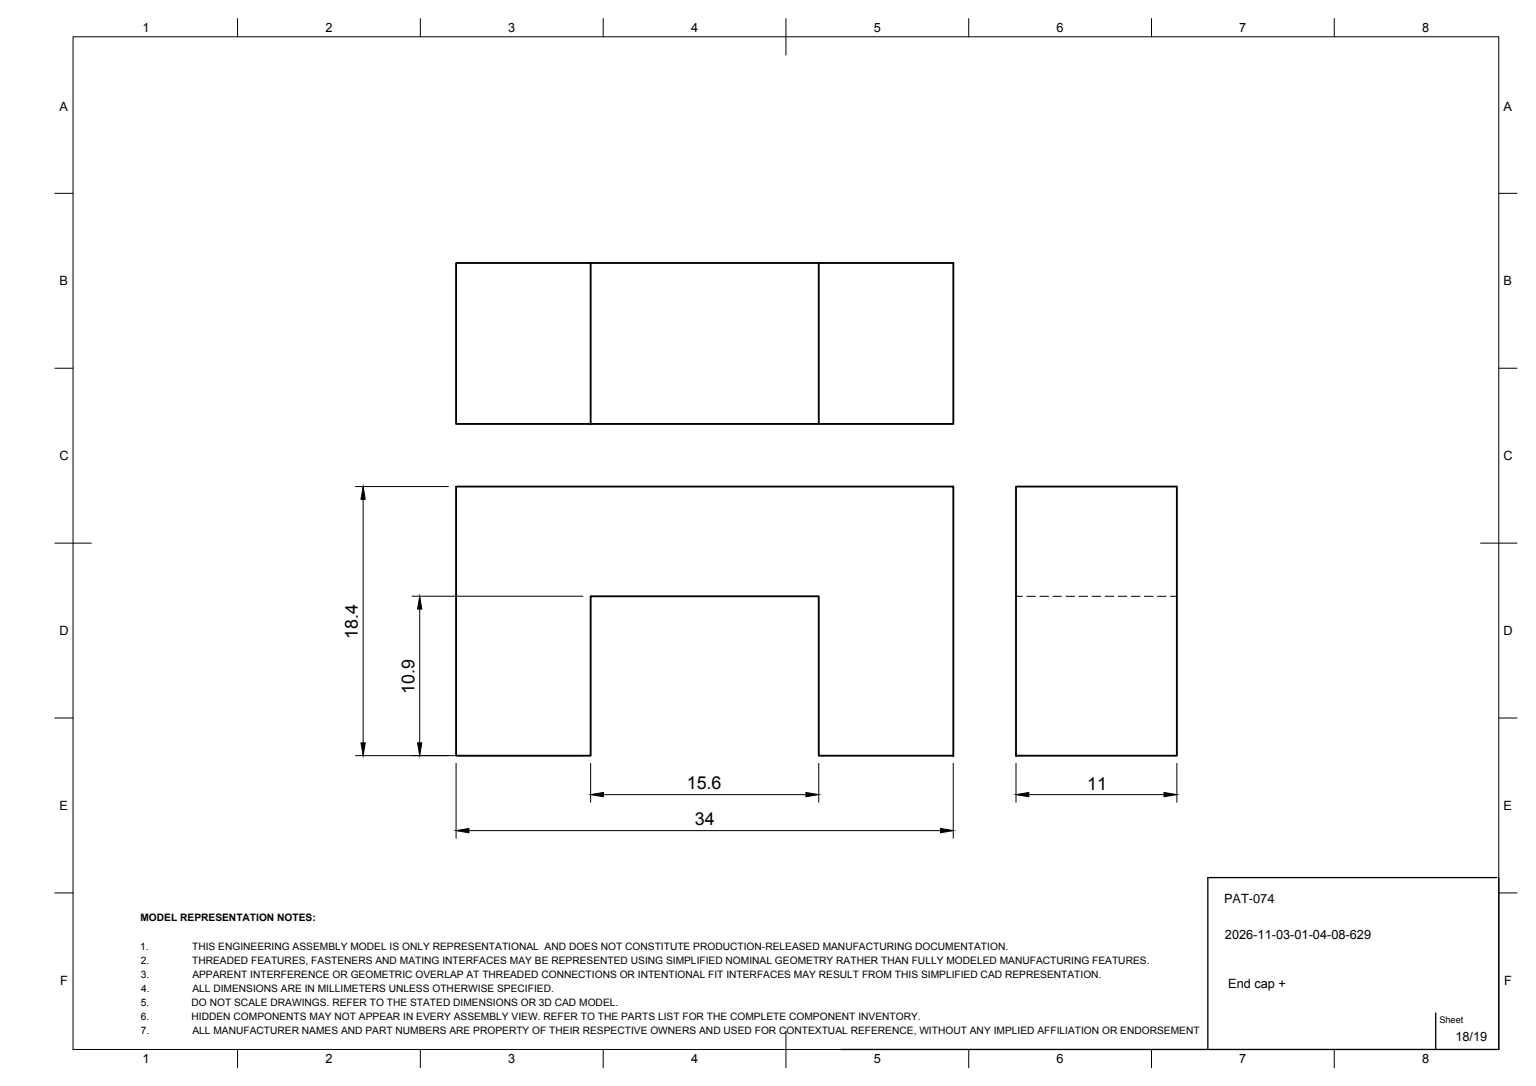
ISO-10303-21;
HEADER;
/* Generated by software containing ST-Developer
 * from STEP Tools, Inc. (www.steptools.com) 
 */

FILE_DESCRIPTION(
/* description */ ('Manual rail carriage with stops'),
/* implementation_level */ '2;1');

FILE_NAME(
/* name */ 'End cap +.step',
/* time_stamp */ '2026-10-27T18:54:27-07:00',
/* author */ (''),
/* organization */ (''),
/* preprocessor_version */ 'ST-DEVELOPER v20.2',
/* originating_system */ 'Autodesk Translation Framework v15.17.0.0',
/* authorisation */ '');

FILE_SCHEMA (('AUTOMOTIVE_DESIGN { 1 0 10303 214 3 1 1 }'));
ENDSEC;

DATA;
#10=MECHANICAL_DESIGN_GEOMETRIC_PRESENTATION_REPRESENTATION('',(#283),#8499);
#247=SHAPE_REPRESENTATION_RELATIONSHIP('SRR','None',#8612,#265);
#265=ADVANCED_BREP_SHAPE_REPRESENTATION('',(#299),#8491);
#283=STYLED_ITEM('',(#8781),#299);
#299=MANIFOLD_SOLID_BREP('Body1',#4953);
#523=PLANE('',#5454);
#524=PLANE('',#5455);
#525=PLANE('',#5456);
#526=PLANE('',#5457);
#527=PLANE('',#5458);
#528=PLANE('',#5459);
#529=PLANE('',#5460);
#530=PLANE('',#5461);
#531=PLANE('',#5462);
#532=PLANE('',#5463);
#763=FACE_OUTER_BOUND('',#1083,.T.);
#764=FACE_OUTER_BOUND('',#1084,.T.);
#765=FACE_OUTER_BOUND('',#1085,.T.);
#766=FACE_OUTER_BOUND('',#1086,.T.);
#767=FACE_OUTER_BOUND('',#1087,.T.);
#768=FACE_OUTER_BOUND('',#1088,.T.);
#769=FACE_OUTER_BOUND('',#1089,.T.);
#770=FACE_OUTER_BOUND('',#1090,.T.);
#771=FACE_OUTER_BOUND('',#1091,.T.);
#772=FACE_OUTER_BOUND('',#1092,.T.);
#1083=EDGE_LOOP('',(#4300,#4301,#4302,#4303));
#1084=EDGE_LOOP('',(#4304,#4305,#4306,#4307));
#1085=EDGE_LOOP('',(#4308,#4309,#4310,#4311));
#1086=EDGE_LOOP('',(#4312,#4313,#4314,#4315));
#1087=EDGE_LOOP('',(#4316,#4317,#4318,#4319));
#1088=EDGE_LOOP('',(#4320,#4321,#4322,#4323));
#1089=EDGE_LOOP('',(#4324,#4325,#4326,#4327));
#1090=EDGE_LOOP('',(#4328,#4329,#4330,#4331));
#1091=EDGE_LOOP('',(#4332,#4333,#4334,#4335,#4336,#4337,#4338,#4339));
#1092=EDGE_LOOP('',(#4340,#4341,#4342,#4343,#4344,#4345,#4346,#4347));
#1561=LINE('',#8054,#2061);
#1562=LINE('',#8056,#2062);
#1563=LINE('',#8058,#2063);
#1564=LINE('',#8059,#2064);
#1565=LINE('',#8062,#2065);
#1566=LINE('',#8064,#2066);
#1567=LINE('',#8065,#2067);
#1568=LINE('',#8068,#2068);
#1569=LINE('',#8070,#2069);
#1570=LINE('',#8071,#2070);
#1571=LINE('',#8074,#2071);
#1572=LINE('',#8076,#2072);
#1573=LINE('',#8077,#2073);
#1574=LINE('',#8080,#2074);
#1575=LINE('',#8082,#2075);
#1576=LINE('',#8083,#2076);
#1577=LINE('',#8086,#2077);
#1578=LINE('',#8088,#2078);
#1579=LINE('',#8089,#2079);
#1580=LINE('',#8092,#2080);
#1581=LINE('',#8094,#2081);
#1582=LINE('',#8095,#2082);
#1583=LINE('',#8097,#2083);
#1584=LINE('',#8098,#2084);
#2061=VECTOR('',#6596,1.);
#2062=VECTOR('',#6597,1.);
#2063=VECTOR('',#6598,1.);
#2064=VECTOR('',#6599,1.);
#2065=VECTOR('',#6602,1.);
#2066=VECTOR('',#6603,1.);
#2067=VECTOR('',#6604,1.);
#2068=VECTOR('',#6607,1.);
#2069=VECTOR('',#6608,1.);
#2070=VECTOR('',#6609,1.);
#2071=VECTOR('',#6612,1.);
#2072=VECTOR('',#6613,1.);
#2073=VECTOR('',#6614,1.);
#2074=VECTOR('',#6617,1.);
#2075=VECTOR('',#6618,1.);
#2076=VECTOR('',#6619,1.);
#2077=VECTOR('',#6622,1.);
#2078=VECTOR('',#6623,1.);
#2079=VECTOR('',#6624,1.);
#2080=VECTOR('',#6627,1.);
#2081=VECTOR('',#6628,1.);
#2082=VECTOR('',#6629,1.);
#2083=VECTOR('',#6632,1.);
#2084=VECTOR('',#6633,1.);
#2623=VERTEX_POINT('',#8052);
#2624=VERTEX_POINT('',#8053);
#2625=VERTEX_POINT('',#8055);
#2626=VERTEX_POINT('',#8057);
#2627=VERTEX_POINT('',#8061);
#2628=VERTEX_POINT('',#8063);
#2629=VERTEX_POINT('',#8067);
#2630=VERTEX_POINT('',#8069);
#2631=VERTEX_POINT('',#8073);
#2632=VERTEX_POINT('',#8075);
#2633=VERTEX_POINT('',#8079);
#2634=VERTEX_POINT('',#8081);
#2635=VERTEX_POINT('',#8085);
#2636=VERTEX_POINT('',#8087);
#2637=VERTEX_POINT('',#8091);
#2638=VERTEX_POINT('',#8093);
#3198=EDGE_CURVE('',#2623,#2624,#1561,.T.);
#3199=EDGE_CURVE('',#2624,#2625,#1562,.T.);
#3200=EDGE_CURVE('',#2626,#2625,#1563,.T.);
#3201=EDGE_CURVE('',#2623,#2626,#1564,.T.);
#3202=EDGE_CURVE('',#2627,#2623,#1565,.T.);
#3203=EDGE_CURVE('',#2628,#2626,#1566,.T.);
#3204=EDGE_CURVE('',#2627,#2628,#1567,.T.);
#3205=EDGE_CURVE('',#2629,#2627,#1568,.T.);
#3206=EDGE_CURVE('',#2630,#2628,#1569,.T.);
#3207=EDGE_CURVE('',#2629,#2630,#1570,.T.);
#3208=EDGE_CURVE('',#2631,#2629,#1571,.T.);
#3209=EDGE_CURVE('',#2632,#2630,#1572,.T.);
#3210=EDGE_CURVE('',#2631,#2632,#1573,.T.);
#3211=EDGE_CURVE('',#2633,#2631,#1574,.T.);
#3212=EDGE_CURVE('',#2634,#2632,#1575,.T.);
#3213=EDGE_CURVE('',#2633,#2634,#1576,.T.);
#3214=EDGE_CURVE('',#2635,#2633,#1577,.T.);
#3215=EDGE_CURVE('',#2636,#2634,#1578,.T.);
#3216=EDGE_CURVE('',#2635,#2636,#1579,.T.);
#3217=EDGE_CURVE('',#2637,#2635,#1580,.T.);
#3218=EDGE_CURVE('',#2638,#2636,#1581,.T.);
#3219=EDGE_CURVE('',#2637,#2638,#1582,.T.);
#3220=EDGE_CURVE('',#2624,#2637,#1583,.T.);
#3221=EDGE_CURVE('',#2625,#2638,#1584,.T.);
#4300=ORIENTED_EDGE('',*,*,#3198,.T.);
#4301=ORIENTED_EDGE('',*,*,#3199,.T.);
#4302=ORIENTED_EDGE('',*,*,#3200,.F.);
#4303=ORIENTED_EDGE('',*,*,#3201,.F.);
#4304=ORIENTED_EDGE('',*,*,#3202,.T.);
#4305=ORIENTED_EDGE('',*,*,#3201,.T.);
#4306=ORIENTED_EDGE('',*,*,#3203,.F.);
#4307=ORIENTED_EDGE('',*,*,#3204,.F.);
#4308=ORIENTED_EDGE('',*,*,#3205,.T.);
#4309=ORIENTED_EDGE('',*,*,#3204,.T.);
#4310=ORIENTED_EDGE('',*,*,#3206,.F.);
#4311=ORIENTED_EDGE('',*,*,#3207,.F.);
#4312=ORIENTED_EDGE('',*,*,#3208,.T.);
#4313=ORIENTED_EDGE('',*,*,#3207,.T.);
#4314=ORIENTED_EDGE('',*,*,#3209,.F.);
#4315=ORIENTED_EDGE('',*,*,#3210,.F.);
#4316=ORIENTED_EDGE('',*,*,#3211,.T.);
#4317=ORIENTED_EDGE('',*,*,#3210,.T.);
#4318=ORIENTED_EDGE('',*,*,#3212,.F.);
#4319=ORIENTED_EDGE('',*,*,#3213,.F.);
#4320=ORIENTED_EDGE('',*,*,#3214,.T.);
#4321=ORIENTED_EDGE('',*,*,#3213,.T.);
#4322=ORIENTED_EDGE('',*,*,#3215,.F.);
#4323=ORIENTED_EDGE('',*,*,#3216,.F.);
#4324=ORIENTED_EDGE('',*,*,#3217,.T.);
#4325=ORIENTED_EDGE('',*,*,#3216,.T.);
#4326=ORIENTED_EDGE('',*,*,#3218,.F.);
#4327=ORIENTED_EDGE('',*,*,#3219,.F.);
#4328=ORIENTED_EDGE('',*,*,#3220,.T.);
#4329=ORIENTED_EDGE('',*,*,#3219,.T.);
#4330=ORIENTED_EDGE('',*,*,#3221,.F.);
#4331=ORIENTED_EDGE('',*,*,#3199,.F.);
#4332=ORIENTED_EDGE('',*,*,#3221,.T.);
#4333=ORIENTED_EDGE('',*,*,#3218,.T.);
#4334=ORIENTED_EDGE('',*,*,#3215,.T.);
#4335=ORIENTED_EDGE('',*,*,#3212,.T.);
#4336=ORIENTED_EDGE('',*,*,#3209,.T.);
#4337=ORIENTED_EDGE('',*,*,#3206,.T.);
#4338=ORIENTED_EDGE('',*,*,#3203,.T.);
#4339=ORIENTED_EDGE('',*,*,#3200,.T.);
#4340=ORIENTED_EDGE('',*,*,#3220,.F.);
#4341=ORIENTED_EDGE('',*,*,#3198,.F.);
#4342=ORIENTED_EDGE('',*,*,#3202,.F.);
#4343=ORIENTED_EDGE('',*,*,#3205,.F.);
#4344=ORIENTED_EDGE('',*,*,#3208,.F.);
#4345=ORIENTED_EDGE('',*,*,#3211,.F.);
#4346=ORIENTED_EDGE('',*,*,#3214,.F.);
#4347=ORIENTED_EDGE('',*,*,#3217,.F.);
#4862=ADVANCED_FACE('',(#763),#523,.T.);
#4863=ADVANCED_FACE('',(#764),#524,.T.);
#4864=ADVANCED_FACE('',(#765),#525,.T.);
#4865=ADVANCED_FACE('',(#766),#526,.T.);
#4866=ADVANCED_FACE('',(#767),#527,.T.);
#4867=ADVANCED_FACE('',(#768),#528,.T.);
#4868=ADVANCED_FACE('',(#769),#529,.T.);
#4869=ADVANCED_FACE('',(#770),#530,.T.);
#4870=ADVANCED_FACE('',(#771),#531,.T.);
#4871=ADVANCED_FACE('',(#772),#532,.F.);
#4953=CLOSED_SHELL('',(#4862,#4863,#4864,#4865,#4866,#4867,#4868,#4869,
#4870,#4871));
#5453=AXIS2_PLACEMENT_3D('',#8050,#6592,#6593);
#5454=AXIS2_PLACEMENT_3D('',#8051,#6594,#6595);
#5455=AXIS2_PLACEMENT_3D('',#8060,#6600,#6601);
#5456=AXIS2_PLACEMENT_3D('',#8066,#6605,#6606);
#5457=AXIS2_PLACEMENT_3D('',#8072,#6610,#6611);
#5458=AXIS2_PLACEMENT_3D('',#8078,#6615,#6616);
#5459=AXIS2_PLACEMENT_3D('',#8084,#6620,#6621);
#5460=AXIS2_PLACEMENT_3D('',#8090,#6625,#6626);
#5461=AXIS2_PLACEMENT_3D('',#8096,#6630,#6631);
#5462=AXIS2_PLACEMENT_3D('',#8099,#6634,#6635);
#5463=AXIS2_PLACEMENT_3D('',#8100,#6636,#6637);
#6592=DIRECTION('axis',(0.,0.,1.));
#6593=DIRECTION('refdir',(1.,0.,0.));
#6594=DIRECTION('center_axis',(0.,0.,1.));
#6595=DIRECTION('ref_axis',(0.,-1.,0.));
#6596=DIRECTION('',(0.,-1.,0.));
#6597=DIRECTION('',(1.,0.,0.));
#6598=DIRECTION('',(0.,-1.,0.));
#6599=DIRECTION('',(1.,0.,0.));
#6600=DIRECTION('center_axis',(0.,1.,0.));
#6601=DIRECTION('ref_axis',(0.,0.,1.));
#6602=DIRECTION('',(0.,0.,1.));
#6603=DIRECTION('',(0.,0.,1.));
#6604=DIRECTION('',(1.,0.,0.));
#6605=DIRECTION('center_axis',(0.,0.,-1.));
#6606=DIRECTION('ref_axis',(0.,1.,0.));
#6607=DIRECTION('',(0.,1.,0.));
#6608=DIRECTION('',(0.,1.,0.));
#6609=DIRECTION('',(1.,0.,0.));
#6610=DIRECTION('center_axis',(0.,-1.,0.));
#6611=DIRECTION('ref_axis',(0.,0.,-1.));
#6612=DIRECTION('',(0.,0.,-1.));
#6613=DIRECTION('',(0.,0.,-1.));
#6614=DIRECTION('',(1.,0.,0.));
#6615=DIRECTION('center_axis',(0.,0.,-1.));
#6616=DIRECTION('ref_axis',(0.,1.,0.));
#6617=DIRECTION('',(0.,1.,0.));
#6618=DIRECTION('',(0.,1.,0.));
#6619=DIRECTION('',(1.,0.,0.));
#6620=DIRECTION('center_axis',(0.,1.,0.));
#6621=DIRECTION('ref_axis',(0.,0.,1.));
#6622=DIRECTION('',(0.,0.,1.));
#6623=DIRECTION('',(0.,0.,1.));
#6624=DIRECTION('',(1.,0.,0.));
#6625=DIRECTION('center_axis',(0.,0.,-1.));
#6626=DIRECTION('ref_axis',(0.,1.,0.));
#6627=DIRECTION('',(0.,1.,0.));
#6628=DIRECTION('',(0.,1.,0.));
#6629=DIRECTION('',(1.,0.,0.));
#6630=DIRECTION('center_axis',(0.,-1.,0.));
#6631=DIRECTION('ref_axis',(0.,0.,-1.));
#6632=DIRECTION('',(0.,0.,-1.));
#6633=DIRECTION('',(0.,0.,-1.));
#6634=DIRECTION('center_axis',(1.,0.,0.));
#6635=DIRECTION('ref_axis',(0.,0.,-1.));
#6636=DIRECTION('center_axis',(1.,0.,0.));
#6637=DIRECTION('ref_axis',(0.,0.,-1.));
#8050=CARTESIAN_POINT('',(0.,0.,0.));
#8051=CARTESIAN_POINT('Origin',(1.97,1.7,2.3));
#8052=CARTESIAN_POINT('',(1.97,1.7,2.3));
#8053=CARTESIAN_POINT('',(1.97,-1.7,2.3));
#8054=CARTESIAN_POINT('',(1.97,1.7,2.3));
#8055=CARTESIAN_POINT('',(3.07,-1.7,2.3));
#8056=CARTESIAN_POINT('',(1.97,-1.7,2.3));
#8057=CARTESIAN_POINT('',(3.07,1.7,2.3));
#8058=CARTESIAN_POINT('',(3.07,1.7,2.3));
#8059=CARTESIAN_POINT('',(1.97,1.7,2.3));
#8060=CARTESIAN_POINT('Origin',(1.97,1.7,0.46));
#8061=CARTESIAN_POINT('',(1.97,1.7,0.46));
#8062=CARTESIAN_POINT('',(1.97,1.7,0.46));
#8063=CARTESIAN_POINT('',(3.07,1.7,0.46));
#8064=CARTESIAN_POINT('',(3.07,1.7,0.46));
#8065=CARTESIAN_POINT('',(1.97,1.7,0.46));
#8066=CARTESIAN_POINT('Origin',(1.97,0.78,0.46));
#8067=CARTESIAN_POINT('',(1.97,0.78,0.46));
#8068=CARTESIAN_POINT('',(1.97,0.78,0.46));
#8069=CARTESIAN_POINT('',(3.07,0.78,0.46));
#8070=CARTESIAN_POINT('',(3.07,0.78,0.46));
#8071=CARTESIAN_POINT('',(1.97,0.78,0.46));
#8072=CARTESIAN_POINT('Origin',(1.97,0.78,1.55));
#8073=CARTESIAN_POINT('',(1.97,0.78,1.55));
#8074=CARTESIAN_POINT('',(1.97,0.78,1.55));
#8075=CARTESIAN_POINT('',(3.07,0.78,1.55));
#8076=CARTESIAN_POINT('',(3.07,0.78,1.55));
#8077=CARTESIAN_POINT('',(1.97,0.78,1.55));
#8078=CARTESIAN_POINT('Origin',(1.97,-0.78,1.55));
#8079=CARTESIAN_POINT('',(1.97,-0.78,1.55));
#8080=CARTESIAN_POINT('',(1.97,-0.78,1.55));
#8081=CARTESIAN_POINT('',(3.07,-0.78,1.55));
#8082=CARTESIAN_POINT('',(3.07,-0.78,1.55));
#8083=CARTESIAN_POINT('',(1.97,-0.78,1.55));
#8084=CARTESIAN_POINT('Origin',(1.97,-0.78,0.46));
#8085=CARTESIAN_POINT('',(1.97,-0.78,0.46));
#8086=CARTESIAN_POINT('',(1.97,-0.78,0.46));
#8087=CARTESIAN_POINT('',(3.07,-0.78,0.46));
#8088=CARTESIAN_POINT('',(3.07,-0.78,0.46));
#8089=CARTESIAN_POINT('',(1.97,-0.78,0.46));
#8090=CARTESIAN_POINT('Origin',(1.97,-1.7,0.46));
#8091=CARTESIAN_POINT('',(1.97,-1.7,0.46));
#8092=CARTESIAN_POINT('',(1.97,-1.7,0.46));
#8093=CARTESIAN_POINT('',(3.07,-1.7,0.46));
#8094=CARTESIAN_POINT('',(3.07,-1.7,0.46));
#8095=CARTESIAN_POINT('',(1.97,-1.7,0.46));
#8096=CARTESIAN_POINT('Origin',(1.97,-1.7,2.3));
#8097=CARTESIAN_POINT('',(1.97,-1.7,2.3));
#8098=CARTESIAN_POINT('',(3.07,-1.7,2.3));
#8099=CARTESIAN_POINT('Origin',(3.07,0.,1.38));
#8100=CARTESIAN_POINT('Origin',(1.97,0.,1.38));
#8468=UNCERTAINTY_MEASURE_WITH_UNIT(LENGTH_MEASURE(0.001),#8500,
'DISTANCE_ACCURACY_VALUE',
'Maximum model space distance between geometric entities at asserted c
onnectivities');
#8476=UNCERTAINTY_MEASURE_WITH_UNIT(LENGTH_MEASURE(0.001),#8500,
'DISTANCE_ACCURACY_VALUE',
'Maximum model space distance between geometric entities at asserted c
onnectivities');
#8491=(
GEOMETRIC_REPRESENTATION_CONTEXT(3)
GLOBAL_UNCERTAINTY_ASSIGNED_CONTEXT((#8468))
GLOBAL_UNIT_ASSIGNED_CONTEXT((#8500,#8502,#8503))
REPRESENTATION_CONTEXT('','3D')
);
#8499=(
GEOMETRIC_REPRESENTATION_CONTEXT(3)
GLOBAL_UNCERTAINTY_ASSIGNED_CONTEXT((#8476))
GLOBAL_UNIT_ASSIGNED_CONTEXT((#8500,#8502,#8503))
REPRESENTATION_CONTEXT('','3D')
);
#8500=(
LENGTH_UNIT()
NAMED_UNIT(*)
SI_UNIT(.CENTI.,.METRE.)
);
#8502=(
NAMED_UNIT(*)
PLANE_ANGLE_UNIT()
SI_UNIT($,.RADIAN.)
);
#8503=(
NAMED_UNIT(*)
SI_UNIT($,.STERADIAN.)
SOLID_ANGLE_UNIT()
);
#8518=SHAPE_DEFINITION_REPRESENTATION(#8540,#8612);
#8540=PRODUCT_DEFINITION_SHAPE('',$,#8635);
#8612=SHAPE_REPRESENTATION('',(#5453),#8491);
#8620=PRODUCT_DEFINITION_CONTEXT('part definition',#8688,'design');
#8635=PRODUCT_DEFINITION('End cap +','End cap +',#8657,#8620);
#8657=PRODUCT_DEFINITION_FORMATION('',$,#8704);
#8688=APPLICATION_CONTEXT(
'Core Data for Automotive Mechanical Design Process');
#8689=PRODUCT_CONTEXT('part definition',#8688,'mechanical');
#8704=PRODUCT('End cap +','End cap +','End cap +',(#8689));
#8775=COLOUR_RGB('Sky Blue',0.24,0.69,0.87);
#8776=FILL_AREA_STYLE_COLOUR('',#8775);
#8777=FILL_AREA_STYLE('',(#8776));
#8778=SURFACE_STYLE_FILL_AREA(#8777);
#8779=SURFACE_SIDE_STYLE('',(#8778));
#8780=SURFACE_STYLE_USAGE(.BOTH.,#8779);
#8781=PRESENTATION_STYLE_ASSIGNMENT((#8780));
ENDSEC;
END-ISO-10303-21;
